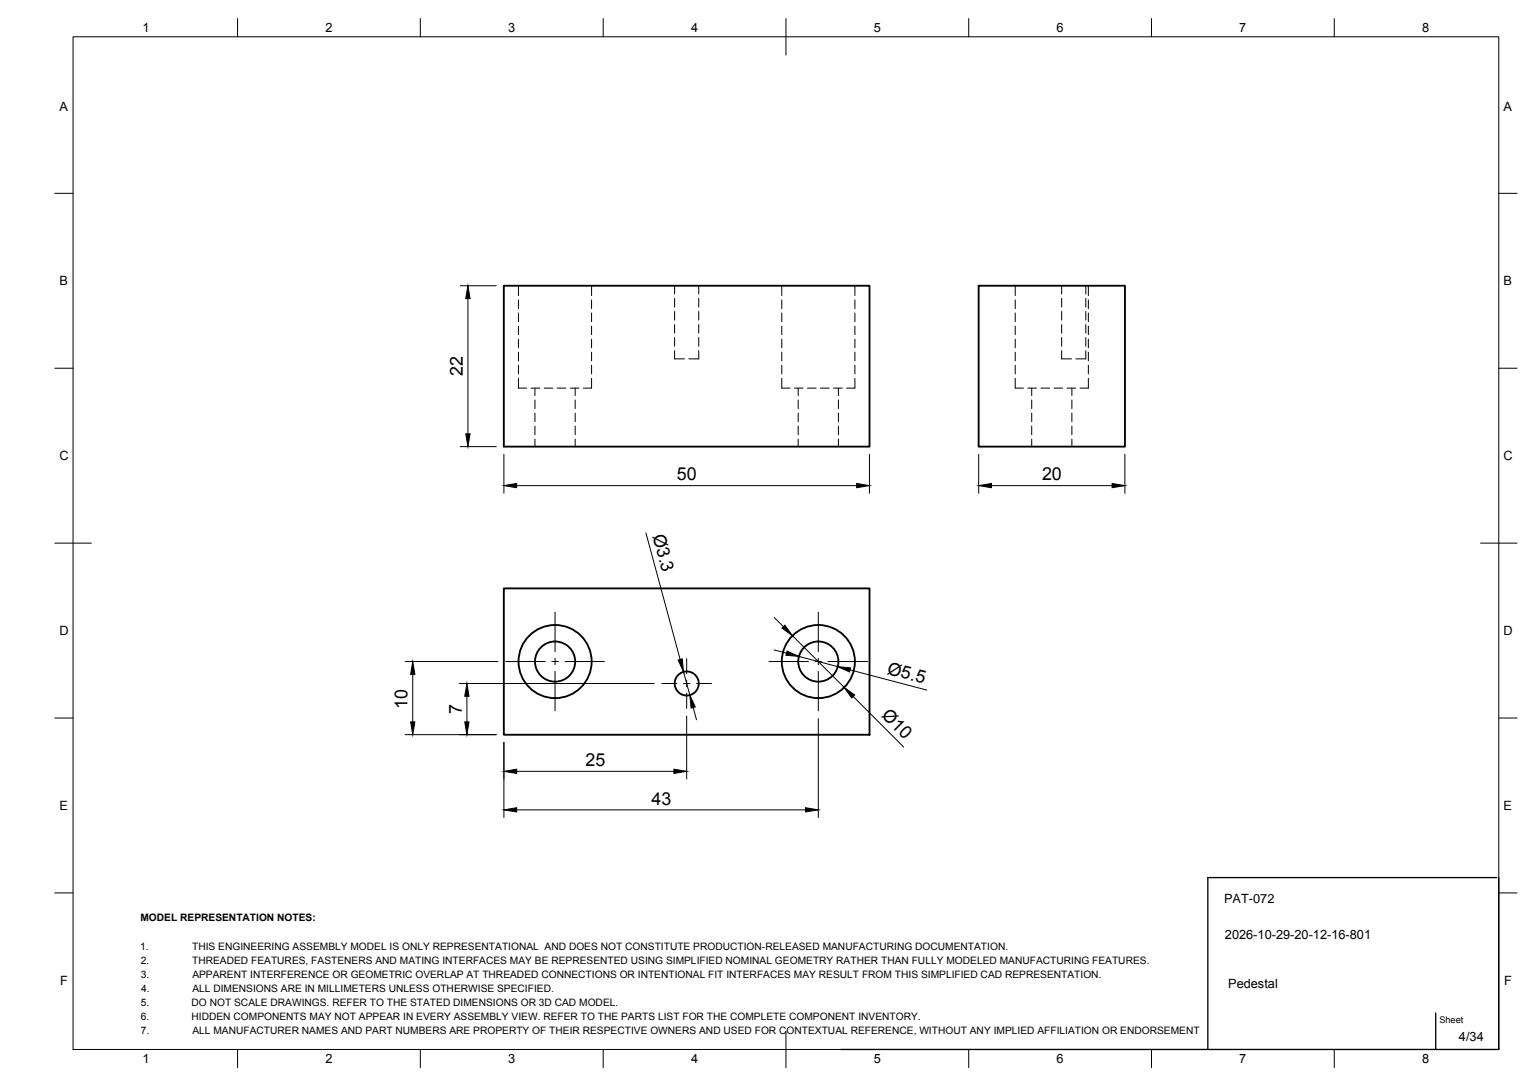
ISO-10303-21;
HEADER;
/* Generated by software containing ST-Developer
 * from STEP Tools, Inc. (www.steptools.com) 
 */

FILE_DESCRIPTION(
/* description */ ('PAT-072'),
/* implementation_level */ '2;1');

FILE_NAME(
/* name */ 'Pedestal.step',
/* time_stamp */ '2026-10-29T20:11:56-07:00',
/* author */ (''),
/* organization */ (''),
/* preprocessor_version */ 'ST-DEVELOPER v20.2',
/* originating_system */ 'Autodesk Translation Framework v15.17.0.0',
/* authorisation */ '');

FILE_SCHEMA (('AUTOMOTIVE_DESIGN { 1 0 10303 214 3 1 1 }'));
ENDSEC;

DATA;
#10=MECHANICAL_DESIGN_GEOMETRIC_PRESENTATION_REPRESENTATION('',(#333),#11432);
#261=SHAPE_REPRESENTATION_RELATIONSHIP('SRR','None',#11565,#297);
#297=ADVANCED_BREP_SHAPE_REPRESENTATION('',(#369),#11396);
#333=STYLED_ITEM('',(#11805),#369);
#369=MANIFOLD_SOLID_BREP('Body1',#6068);
#410=FACE_BOUND('',#1190,.T.);
#411=FACE_BOUND('',#1193,.T.);
#412=FACE_BOUND('',#1201,.T.);
#413=FACE_BOUND('',#1202,.T.);
#414=FACE_BOUND('',#1203,.T.);
#415=FACE_BOUND('',#1205,.T.);
#416=FACE_BOUND('',#1206,.T.);
#576=PLANE('',#6526);
#577=PLANE('',#6530);
#578=PLANE('',#6535);
#579=PLANE('',#6541);
#580=PLANE('',#6542);
#581=PLANE('',#6543);
#582=PLANE('',#6544);
#583=PLANE('',#6545);
#584=PLANE('',#6546);
#806=FACE_OUTER_BOUND('',#1186,.T.);
#807=FACE_OUTER_BOUND('',#1187,.T.);
#808=FACE_OUTER_BOUND('',#1188,.T.);
#809=FACE_OUTER_BOUND('',#1189,.T.);
#810=FACE_OUTER_BOUND('',#1191,.T.);
#811=FACE_OUTER_BOUND('',#1192,.T.);
#812=FACE_OUTER_BOUND('',#1194,.T.);
#813=FACE_OUTER_BOUND('',#1195,.T.);
#814=FACE_OUTER_BOUND('',#1196,.T.);
#815=FACE_OUTER_BOUND('',#1197,.T.);
#816=FACE_OUTER_BOUND('',#1198,.T.);
#817=FACE_OUTER_BOUND('',#1199,.T.);
#818=FACE_OUTER_BOUND('',#1200,.T.);
#819=FACE_OUTER_BOUND('',#1204,.T.);
#1186=EDGE_LOOP('',(#4116,#4117,#4118,#4119));
#1187=EDGE_LOOP('',(#4120));
#1188=EDGE_LOOP('',(#4121,#4122,#4123,#4124));
#1189=EDGE_LOOP('',(#4125));
#1190=EDGE_LOOP('',(#4126));
#1191=EDGE_LOOP('',(#4127,#4128,#4129,#4130));
#1192=EDGE_LOOP('',(#4131));
#1193=EDGE_LOOP('',(#4132));
#1194=EDGE_LOOP('',(#4133,#4134,#4135,#4136));
#1195=EDGE_LOOP('',(#4137,#4138,#4139,#4140));
#1196=EDGE_LOOP('',(#4141,#4142,#4143,#4144));
#1197=EDGE_LOOP('',(#4145,#4146,#4147,#4148));
#1198=EDGE_LOOP('',(#4149,#4150,#4151,#4152));
#1199=EDGE_LOOP('',(#4153,#4154,#4155,#4156));
#1200=EDGE_LOOP('',(#4157,#4158,#4159,#4160));
#1201=EDGE_LOOP('',(#4161));
#1202=EDGE_LOOP('',(#4162));
#1203=EDGE_LOOP('',(#4163));
#1204=EDGE_LOOP('',(#4164,#4165,#4166,#4167));
#1205=EDGE_LOOP('',(#4168));
#1206=EDGE_LOOP('',(#4169));
#1724=LINE('',#9249,#2143);
#1725=LINE('',#9256,#2144);
#1726=LINE('',#9265,#2145);
#1727=LINE('',#9273,#2146);
#1728=LINE('',#9277,#2147);
#1729=LINE('',#9281,#2148);
#1730=LINE('',#9283,#2149);
#1731=LINE('',#9285,#2150);
#1732=LINE('',#9286,#2151);
#1733=LINE('',#9289,#2152);
#1734=LINE('',#9291,#2153);
#1735=LINE('',#9292,#2154);
#1736=LINE('',#9295,#2155);
#1737=LINE('',#9297,#2156);
#1738=LINE('',#9298,#2157);
#1739=LINE('',#9300,#2158);
#1740=LINE('',#9301,#2159);
#2143=VECTOR('',#7321,0.165);
#2144=VECTOR('',#7330,0.5);
#2145=VECTOR('',#7341,0.5);
#2146=VECTOR('',#7352,0.275);
#2147=VECTOR('',#7357,0.275);
#2148=VECTOR('',#7360,1.);
#2149=VECTOR('',#7361,1.);
#2150=VECTOR('',#7362,1.);
#2151=VECTOR('',#7363,1.);
#2152=VECTOR('',#7366,1.);
#2153=VECTOR('',#7367,1.);
#2154=VECTOR('',#7368,1.);
#2155=VECTOR('',#7371,1.);
#2156=VECTOR('',#7372,1.);
#2157=VECTOR('',#7373,1.);
#2158=VECTOR('',#7376,1.);
#2159=VECTOR('',#7377,1.);
#2554=CIRCLE('',#6524,0.165);
#2555=CIRCLE('',#6525,0.165);
#2556=CIRCLE('',#6528,0.5);
#2557=CIRCLE('',#6529,0.5);
#2558=CIRCLE('',#6531,0.275);
#2559=CIRCLE('',#6533,0.5);
#2560=CIRCLE('',#6534,0.5);
#2561=CIRCLE('',#6536,0.275);
#2562=CIRCLE('',#6538,0.275);
#2563=CIRCLE('',#6540,0.275);
#2852=VERTEX_POINT('',#9246);
#2853=VERTEX_POINT('',#9248);
#2854=VERTEX_POINT('',#9253);
#2855=VERTEX_POINT('',#9255);
#2856=VERTEX_POINT('',#9259);
#2857=VERTEX_POINT('',#9262);
#2858=VERTEX_POINT('',#9264);
#2859=VERTEX_POINT('',#9268);
#2860=VERTEX_POINT('',#9271);
#2861=VERTEX_POINT('',#9275);
#2862=VERTEX_POINT('',#9279);
#2863=VERTEX_POINT('',#9280);
#2864=VERTEX_POINT('',#9282);
#2865=VERTEX_POINT('',#9284);
#2866=VERTEX_POINT('',#9288);
#2867=VERTEX_POINT('',#9290);
#2868=VERTEX_POINT('',#9294);
#2869=VERTEX_POINT('',#9296);
#3347=EDGE_CURVE('',#2852,#2852,#2554,.T.);
#3348=EDGE_CURVE('',#2852,#2853,#1724,.T.);
#3349=EDGE_CURVE('',#2853,#2853,#2555,.T.);
#3350=EDGE_CURVE('',#2854,#2854,#2556,.T.);
#3351=EDGE_CURVE('',#2854,#2855,#1725,.T.);
#3352=EDGE_CURVE('',#2855,#2855,#2557,.T.);
#3353=EDGE_CURVE('',#2856,#2856,#2558,.T.);
#3354=EDGE_CURVE('',#2857,#2857,#2559,.T.);
#3355=EDGE_CURVE('',#2857,#2858,#1726,.T.);
#3356=EDGE_CURVE('',#2858,#2858,#2560,.T.);
#3357=EDGE_CURVE('',#2859,#2859,#2561,.T.);
#3358=EDGE_CURVE('',#2860,#2860,#2562,.T.);
#3359=EDGE_CURVE('',#2860,#2856,#1727,.T.);
#3360=EDGE_CURVE('',#2861,#2861,#2563,.T.);
#3361=EDGE_CURVE('',#2861,#2859,#1728,.T.);
#3362=EDGE_CURVE('',#2862,#2863,#1729,.T.);
#3363=EDGE_CURVE('',#2863,#2864,#1730,.T.);
#3364=EDGE_CURVE('',#2865,#2864,#1731,.T.);
#3365=EDGE_CURVE('',#2862,#2865,#1732,.T.);
#3366=EDGE_CURVE('',#2866,#2862,#1733,.T.);
#3367=EDGE_CURVE('',#2867,#2865,#1734,.T.);
#3368=EDGE_CURVE('',#2866,#2867,#1735,.T.);
#3369=EDGE_CURVE('',#2868,#2866,#1736,.T.);
#3370=EDGE_CURVE('',#2869,#2867,#1737,.T.);
#3371=EDGE_CURVE('',#2868,#2869,#1738,.T.);
#3372=EDGE_CURVE('',#2863,#2868,#1739,.T.);
#3373=EDGE_CURVE('',#2864,#2869,#1740,.T.);
#4116=ORIENTED_EDGE('',*,*,#3347,.F.);
#4117=ORIENTED_EDGE('',*,*,#3348,.T.);
#4118=ORIENTED_EDGE('',*,*,#3349,.F.);
#4119=ORIENTED_EDGE('',*,*,#3348,.F.);
#4120=ORIENTED_EDGE('',*,*,#3347,.T.);
#4121=ORIENTED_EDGE('',*,*,#3350,.F.);
#4122=ORIENTED_EDGE('',*,*,#3351,.T.);
#4123=ORIENTED_EDGE('',*,*,#3352,.F.);
#4124=ORIENTED_EDGE('',*,*,#3351,.F.);
#4125=ORIENTED_EDGE('',*,*,#3350,.T.);
#4126=ORIENTED_EDGE('',*,*,#3353,.F.);
#4127=ORIENTED_EDGE('',*,*,#3354,.F.);
#4128=ORIENTED_EDGE('',*,*,#3355,.T.);
#4129=ORIENTED_EDGE('',*,*,#3356,.F.);
#4130=ORIENTED_EDGE('',*,*,#3355,.F.);
#4131=ORIENTED_EDGE('',*,*,#3354,.T.);
#4132=ORIENTED_EDGE('',*,*,#3357,.F.);
#4133=ORIENTED_EDGE('',*,*,#3358,.F.);
#4134=ORIENTED_EDGE('',*,*,#3359,.T.);
#4135=ORIENTED_EDGE('',*,*,#3353,.T.);
#4136=ORIENTED_EDGE('',*,*,#3359,.F.);
#4137=ORIENTED_EDGE('',*,*,#3360,.F.);
#4138=ORIENTED_EDGE('',*,*,#3361,.T.);
#4139=ORIENTED_EDGE('',*,*,#3357,.T.);
#4140=ORIENTED_EDGE('',*,*,#3361,.F.);
#4141=ORIENTED_EDGE('',*,*,#3362,.T.);
#4142=ORIENTED_EDGE('',*,*,#3363,.T.);
#4143=ORIENTED_EDGE('',*,*,#3364,.F.);
#4144=ORIENTED_EDGE('',*,*,#3365,.F.);
#4145=ORIENTED_EDGE('',*,*,#3366,.T.);
#4146=ORIENTED_EDGE('',*,*,#3365,.T.);
#4147=ORIENTED_EDGE('',*,*,#3367,.F.);
#4148=ORIENTED_EDGE('',*,*,#3368,.F.);
#4149=ORIENTED_EDGE('',*,*,#3369,.T.);
#4150=ORIENTED_EDGE('',*,*,#3368,.T.);
#4151=ORIENTED_EDGE('',*,*,#3370,.F.);
#4152=ORIENTED_EDGE('',*,*,#3371,.F.);
#4153=ORIENTED_EDGE('',*,*,#3372,.T.);
#4154=ORIENTED_EDGE('',*,*,#3371,.T.);
#4155=ORIENTED_EDGE('',*,*,#3373,.F.);
#4156=ORIENTED_EDGE('',*,*,#3363,.F.);
#4157=ORIENTED_EDGE('',*,*,#3373,.T.);
#4158=ORIENTED_EDGE('',*,*,#3370,.T.);
#4159=ORIENTED_EDGE('',*,*,#3367,.T.);
#4160=ORIENTED_EDGE('',*,*,#3364,.T.);
#4161=ORIENTED_EDGE('',*,*,#3349,.T.);
#4162=ORIENTED_EDGE('',*,*,#3352,.T.);
#4163=ORIENTED_EDGE('',*,*,#3356,.T.);
#4164=ORIENTED_EDGE('',*,*,#3372,.F.);
#4165=ORIENTED_EDGE('',*,*,#3362,.F.);
#4166=ORIENTED_EDGE('',*,*,#3366,.F.);
#4167=ORIENTED_EDGE('',*,*,#3369,.F.);
#4168=ORIENTED_EDGE('',*,*,#3358,.T.);
#4169=ORIENTED_EDGE('',*,*,#3360,.T.);
#5562=CYLINDRICAL_SURFACE('',#6523,0.165);
#5563=CYLINDRICAL_SURFACE('',#6527,0.5);
#5564=CYLINDRICAL_SURFACE('',#6532,0.5);
#5565=CYLINDRICAL_SURFACE('',#6537,0.275);
#5566=CYLINDRICAL_SURFACE('',#6539,0.275);
#5705=ADVANCED_FACE('',(#806),#5562,.F.);
#5706=ADVANCED_FACE('',(#807),#576,.T.);
#5707=ADVANCED_FACE('',(#808),#5563,.F.);
#5708=ADVANCED_FACE('',(#809,#410),#577,.T.);
#5709=ADVANCED_FACE('',(#810),#5564,.F.);
#5710=ADVANCED_FACE('',(#811,#411),#578,.T.);
#5711=ADVANCED_FACE('',(#812),#5565,.F.);
#5712=ADVANCED_FACE('',(#813),#5566,.F.);
#5713=ADVANCED_FACE('',(#814),#579,.T.);
#5714=ADVANCED_FACE('',(#815),#580,.T.);
#5715=ADVANCED_FACE('',(#816),#581,.T.);
#5716=ADVANCED_FACE('',(#817),#582,.T.);
#5717=ADVANCED_FACE('',(#818,#412,#413,#414),#583,.T.);
#5718=ADVANCED_FACE('',(#819,#415,#416),#584,.F.);
#6068=CLOSED_SHELL('',(#5705,#5706,#5707,#5708,#5709,#5710,#5711,#5712,
#5713,#5714,#5715,#5716,#5717,#5718));
#6522=AXIS2_PLACEMENT_3D('',#9244,#7315,#7316);
#6523=AXIS2_PLACEMENT_3D('',#9245,#7317,#7318);
#6524=AXIS2_PLACEMENT_3D('',#9247,#7319,#7320);
#6525=AXIS2_PLACEMENT_3D('',#9250,#7322,#7323);
#6526=AXIS2_PLACEMENT_3D('',#9251,#7324,#7325);
#6527=AXIS2_PLACEMENT_3D('',#9252,#7326,#7327);
#6528=AXIS2_PLACEMENT_3D('',#9254,#7328,#7329);
#6529=AXIS2_PLACEMENT_3D('',#9257,#7331,#7332);
#6530=AXIS2_PLACEMENT_3D('',#9258,#7333,#7334);
#6531=AXIS2_PLACEMENT_3D('',#9260,#7335,#7336);
#6532=AXIS2_PLACEMENT_3D('',#9261,#7337,#7338);
#6533=AXIS2_PLACEMENT_3D('',#9263,#7339,#7340);
#6534=AXIS2_PLACEMENT_3D('',#9266,#7342,#7343);
#6535=AXIS2_PLACEMENT_3D('',#9267,#7344,#7345);
#6536=AXIS2_PLACEMENT_3D('',#9269,#7346,#7347);
#6537=AXIS2_PLACEMENT_3D('',#9270,#7348,#7349);
#6538=AXIS2_PLACEMENT_3D('',#9272,#7350,#7351);
#6539=AXIS2_PLACEMENT_3D('',#9274,#7353,#7354);
#6540=AXIS2_PLACEMENT_3D('',#9276,#7355,#7356);
#6541=AXIS2_PLACEMENT_3D('',#9278,#7358,#7359);
#6542=AXIS2_PLACEMENT_3D('',#9287,#7364,#7365);
#6543=AXIS2_PLACEMENT_3D('',#9293,#7369,#7370);
#6544=AXIS2_PLACEMENT_3D('',#9299,#7374,#7375);
#6545=AXIS2_PLACEMENT_3D('',#9302,#7378,#7379);
#6546=AXIS2_PLACEMENT_3D('',#9303,#7380,#7381);
#7315=DIRECTION('axis',(0.,0.,1.));
#7316=DIRECTION('refdir',(1.,0.,0.));
#7317=DIRECTION('center_axis',(0.,0.,1.));
#7318=DIRECTION('ref_axis',(1.,0.,0.));
#7319=DIRECTION('center_axis',(0.,0.,1.));
#7320=DIRECTION('ref_axis',(1.,0.,0.));
#7321=DIRECTION('',(0.,0.,1.));
#7322=DIRECTION('center_axis',(0.,0.,-1.));
#7323=DIRECTION('ref_axis',(1.,0.,0.));
#7324=DIRECTION('center_axis',(0.,0.,1.));
#7325=DIRECTION('ref_axis',(1.,0.,0.));
#7326=DIRECTION('center_axis',(0.,0.,1.));
#7327=DIRECTION('ref_axis',(1.,0.,0.));
#7328=DIRECTION('center_axis',(0.,0.,1.));
#7329=DIRECTION('ref_axis',(1.,0.,0.));
#7330=DIRECTION('',(0.,0.,1.));
#7331=DIRECTION('center_axis',(0.,0.,-1.));
#7332=DIRECTION('ref_axis',(1.,0.,0.));
#7333=DIRECTION('center_axis',(0.,0.,1.));
#7334=DIRECTION('ref_axis',(1.,0.,0.));
#7335=DIRECTION('center_axis',(0.,0.,1.));
#7336=DIRECTION('ref_axis',(1.,0.,0.));
#7337=DIRECTION('center_axis',(0.,0.,1.));
#7338=DIRECTION('ref_axis',(1.,0.,0.));
#7339=DIRECTION('center_axis',(0.,0.,1.));
#7340=DIRECTION('ref_axis',(1.,0.,0.));
#7341=DIRECTION('',(0.,0.,1.));
#7342=DIRECTION('center_axis',(0.,0.,-1.));
#7343=DIRECTION('ref_axis',(1.,0.,0.));
#7344=DIRECTION('center_axis',(0.,0.,1.));
#7345=DIRECTION('ref_axis',(1.,0.,0.));
#7346=DIRECTION('center_axis',(0.,0.,1.));
#7347=DIRECTION('ref_axis',(1.,0.,0.));
#7348=DIRECTION('center_axis',(0.,0.,1.));
#7349=DIRECTION('ref_axis',(1.,0.,0.));
#7350=DIRECTION('center_axis',(0.,0.,1.));
#7351=DIRECTION('ref_axis',(1.,0.,0.));
#7352=DIRECTION('',(0.,0.,1.));
#7353=DIRECTION('center_axis',(0.,0.,1.));
#7354=DIRECTION('ref_axis',(1.,0.,0.));
#7355=DIRECTION('center_axis',(0.,0.,1.));
#7356=DIRECTION('ref_axis',(1.,0.,0.));
#7357=DIRECTION('',(0.,0.,1.));
#7358=DIRECTION('center_axis',(0.,1.,0.));
#7359=DIRECTION('ref_axis',(-1.,0.,0.));
#7360=DIRECTION('',(-1.,0.,0.));
#7361=DIRECTION('',(0.,0.,1.));
#7362=DIRECTION('',(-1.,0.,0.));
#7363=DIRECTION('',(0.,0.,1.));
#7364=DIRECTION('center_axis',(1.,0.,0.));
#7365=DIRECTION('ref_axis',(0.,1.,0.));
#7366=DIRECTION('',(0.,1.,0.));
#7367=DIRECTION('',(0.,1.,0.));
#7368=DIRECTION('',(0.,0.,1.));
#7369=DIRECTION('center_axis',(0.,-1.,0.));
#7370=DIRECTION('ref_axis',(1.,0.,0.));
#7371=DIRECTION('',(1.,0.,0.));
#7372=DIRECTION('',(1.,0.,0.));
#7373=DIRECTION('',(0.,0.,1.));
#7374=DIRECTION('center_axis',(-1.,0.,0.));
#7375=DIRECTION('ref_axis',(0.,-1.,0.));
#7376=DIRECTION('',(0.,-1.,0.));
#7377=DIRECTION('',(0.,-1.,0.));
#7378=DIRECTION('center_axis',(0.,0.,1.));
#7379=DIRECTION('ref_axis',(1.,0.,0.));
#7380=DIRECTION('center_axis',(0.,0.,1.));
#7381=DIRECTION('ref_axis',(1.,0.,0.));
#9244=CARTESIAN_POINT('',(0.,0.,0.));
#9245=CARTESIAN_POINT('Origin',(-4.8,0.,2.));
#9246=CARTESIAN_POINT('',(-4.965,-2.02066721859313E-17,2.));
#9247=CARTESIAN_POINT('Origin',(-4.8,0.,2.));
#9248=CARTESIAN_POINT('',(-4.965,2.02066721859313E-17,3.));
#9249=CARTESIAN_POINT('',(-4.965,-2.02066721859313E-17,2.));
#9250=CARTESIAN_POINT('Origin',(-4.8,0.,3.));
#9251=CARTESIAN_POINT('Origin',(-4.8,0.,2.));
#9252=CARTESIAN_POINT('Origin',(-4.5,-1.8,1.6));
#9253=CARTESIAN_POINT('',(-5.,-1.8,1.6));
#9254=CARTESIAN_POINT('Origin',(-4.5,-1.8,1.6));
#9255=CARTESIAN_POINT('',(-5.,-1.8,3.));
#9256=CARTESIAN_POINT('',(-5.,-1.8,1.6));
#9257=CARTESIAN_POINT('Origin',(-4.5,-1.8,3.));
#9258=CARTESIAN_POINT('Origin',(-4.5,-1.8,1.6));
#9259=CARTESIAN_POINT('',(-4.775,-1.8,1.6));
#9260=CARTESIAN_POINT('Origin',(-4.5,-1.8,1.6));
#9261=CARTESIAN_POINT('Origin',(-4.5,1.8,1.6));
#9262=CARTESIAN_POINT('',(-5.,1.8,1.6));
#9263=CARTESIAN_POINT('Origin',(-4.5,1.8,1.6));
#9264=CARTESIAN_POINT('',(-5.,1.8,3.));
#9265=CARTESIAN_POINT('',(-5.,1.8,1.6));
#9266=CARTESIAN_POINT('Origin',(-4.5,1.8,3.));
#9267=CARTESIAN_POINT('Origin',(-4.5,1.8,1.6));
#9268=CARTESIAN_POINT('',(-4.775,1.8,1.6));
#9269=CARTESIAN_POINT('Origin',(-4.5,1.8,1.6));
#9270=CARTESIAN_POINT('Origin',(-4.5,-1.8,0.7));
#9271=CARTESIAN_POINT('',(-4.775,-1.8,0.8));
#9272=CARTESIAN_POINT('Origin',(-4.5,-1.8,0.8));
#9273=CARTESIAN_POINT('',(-4.775,-1.8,0.7));
#9274=CARTESIAN_POINT('Origin',(-4.5,1.8,0.7));
#9275=CARTESIAN_POINT('',(-4.775,1.8,0.8));
#9276=CARTESIAN_POINT('Origin',(-4.5,1.8,0.8));
#9277=CARTESIAN_POINT('',(-4.775,1.8,0.7));
#9278=CARTESIAN_POINT('Origin',(-3.5,2.5,0.8));
#9279=CARTESIAN_POINT('',(-3.5,2.5,0.8));
#9280=CARTESIAN_POINT('',(-5.5,2.5,0.8));
#9281=CARTESIAN_POINT('',(-3.5,2.5,0.8));
#9282=CARTESIAN_POINT('',(-5.5,2.5,3.));
#9283=CARTESIAN_POINT('',(-5.5,2.5,0.8));
#9284=CARTESIAN_POINT('',(-3.5,2.5,3.));
#9285=CARTESIAN_POINT('',(-3.5,2.5,3.));
#9286=CARTESIAN_POINT('',(-3.5,2.5,0.8));
#9287=CARTESIAN_POINT('Origin',(-3.5,-2.5,0.8));
#9288=CARTESIAN_POINT('',(-3.5,-2.5,0.8));
#9289=CARTESIAN_POINT('',(-3.5,-2.5,0.8));
#9290=CARTESIAN_POINT('',(-3.5,-2.5,3.));
#9291=CARTESIAN_POINT('',(-3.5,-2.5,3.));
#9292=CARTESIAN_POINT('',(-3.5,-2.5,0.8));
#9293=CARTESIAN_POINT('Origin',(-5.5,-2.5,0.8));
#9294=CARTESIAN_POINT('',(-5.5,-2.5,0.8));
#9295=CARTESIAN_POINT('',(-5.5,-2.5,0.8));
#9296=CARTESIAN_POINT('',(-5.5,-2.5,3.));
#9297=CARTESIAN_POINT('',(-5.5,-2.5,3.));
#9298=CARTESIAN_POINT('',(-5.5,-2.5,0.8));
#9299=CARTESIAN_POINT('Origin',(-5.5,2.5,0.8));
#9300=CARTESIAN_POINT('',(-5.5,2.5,0.8));
#9301=CARTESIAN_POINT('',(-5.5,2.5,3.));
#9302=CARTESIAN_POINT('Origin',(-4.5,0.,3.));
#9303=CARTESIAN_POINT('Origin',(-4.5,0.,0.8));
#11357=UNCERTAINTY_MEASURE_WITH_UNIT(LENGTH_MEASURE(0.001),#11433,
'DISTANCE_ACCURACY_VALUE',
'Maximum model space distance between geometric entities at asserted c
onnectivities');
#11393=UNCERTAINTY_MEASURE_WITH_UNIT(LENGTH_MEASURE(0.001),#11433,
'DISTANCE_ACCURACY_VALUE',
'Maximum model space distance between geometric entities at asserted c
onnectivities');
#11396=(
GEOMETRIC_REPRESENTATION_CONTEXT(3)
GLOBAL_UNCERTAINTY_ASSIGNED_CONTEXT((#11357))
GLOBAL_UNIT_ASSIGNED_CONTEXT((#11433,#11435,#11436))
REPRESENTATION_CONTEXT('','3D')
);
#11432=(
GEOMETRIC_REPRESENTATION_CONTEXT(3)
GLOBAL_UNCERTAINTY_ASSIGNED_CONTEXT((#11393))
GLOBAL_UNIT_ASSIGNED_CONTEXT((#11433,#11435,#11436))
REPRESENTATION_CONTEXT('','3D')
);
#11433=(
LENGTH_UNIT()
NAMED_UNIT(*)
SI_UNIT(.CENTI.,.METRE.)
);
#11435=(
NAMED_UNIT(*)
PLANE_ANGLE_UNIT()
SI_UNIT($,.RADIAN.)
);
#11436=(
NAMED_UNIT(*)
SI_UNIT($,.STERADIAN.)
SOLID_ANGLE_UNIT()
);
#11439=SHAPE_DEFINITION_REPRESENTATION(#11477,#11565);
#11477=PRODUCT_DEFINITION_SHAPE('',$,#11604);
#11565=SHAPE_REPRESENTATION('',(#6522),#11396);
#11601=PRODUCT_DEFINITION_CONTEXT('part definition',#11717,'design');
#11604=PRODUCT_DEFINITION('Pedestal','Pedestal',#11642,#11601);
#11642=PRODUCT_DEFINITION_FORMATION('',$,#11721);
#11717=APPLICATION_CONTEXT(
'Core Data for Automotive Mechanical Design Process');
#11718=PRODUCT_CONTEXT('part definition',#11717,'mechanical');
#11721=PRODUCT('Pedestal','Pedestal','Pedestal',(#11718));
#11799=COLOUR_RGB('Light Blue',0.38,0.62,0.78);
#11800=FILL_AREA_STYLE_COLOUR('',#11799);
#11801=FILL_AREA_STYLE('',(#11800));
#11802=SURFACE_STYLE_FILL_AREA(#11801);
#11803=SURFACE_SIDE_STYLE('',(#11802));
#11804=SURFACE_STYLE_USAGE(.BOTH.,#11803);
#11805=PRESENTATION_STYLE_ASSIGNMENT((#11804));
ENDSEC;
END-ISO-10303-21;
